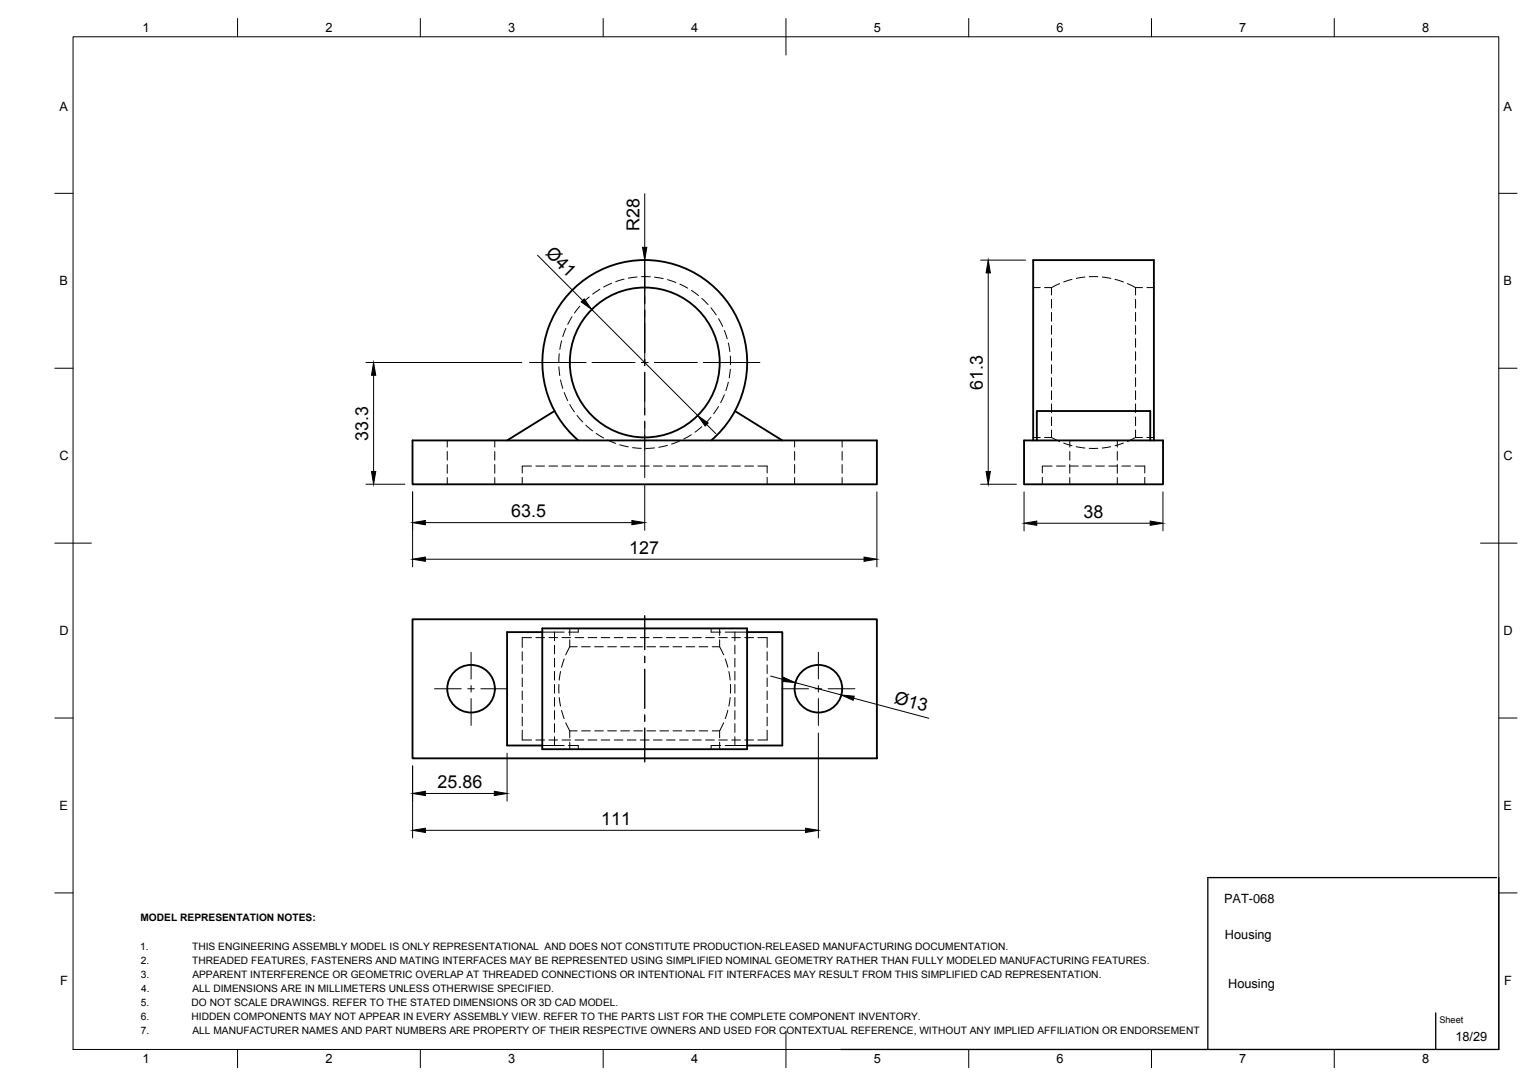
ISO-10303-21;
HEADER;
/* Generated by software containing ST-Developer
 * from STEP Tools, Inc. (www.steptools.com) 
 */

FILE_DESCRIPTION(
/* description */ ('Line shaft on three pillow blocks'),
/* implementation_level */ '2;1');

FILE_NAME(
/* name */ 'Housing.step',
/* time_stamp */ '2026-10-27T10:49:19-07:00',
/* author */ (''),
/* organization */ (''),
/* preprocessor_version */ 'ST-DEVELOPER v20.2',
/* originating_system */ 'Autodesk Translation Framework v15.17.0.0',
/* authorisation */ '');

FILE_SCHEMA (('AUTOMOTIVE_DESIGN { 1 0 10303 214 3 1 1 }'));
ENDSEC;

DATA;
#10=MECHANICAL_DESIGN_GEOMETRIC_PRESENTATION_REPRESENTATION('',(#351),#8377);
#263=SPHERICAL_SURFACE('',#4833,2.35);
#297=SHAPE_REPRESENTATION_RELATIONSHIP('SRR','None',#8513,#324);
#324=ADVANCED_BREP_SHAPE_REPRESENTATION('',(#378),#8362);
#351=STYLED_ITEM('',(#8697),#378);
#378=MANIFOLD_SOLID_BREP('Body1',#4338);
#430=FACE_BOUND('',#1041,.T.);
#431=FACE_BOUND('',#1042,.T.);
#432=FACE_BOUND('',#1050,.T.);
#433=FACE_BOUND('',#1051,.T.);
#434=FACE_BOUND('',#1052,.T.);
#435=FACE_BOUND('',#1055,.T.);
#436=FACE_BOUND('',#1057,.T.);
#437=FACE_BOUND('',#1070,.T.);
#438=FACE_BOUND('',#1071,.T.);
#439=FACE_BOUND('',#1072,.T.);
#547=PLANE('',#4835);
#548=PLANE('',#4837);
#549=PLANE('',#4839);
#550=PLANE('',#4841);
#551=PLANE('',#4842);
#552=PLANE('',#4844);
#553=PLANE('',#4845);
#554=PLANE('',#4851);
#555=PLANE('',#4852);
#556=PLANE('',#4853);
#557=PLANE('',#4854);
#558=PLANE('',#4855);
#559=PLANE('',#4856);
#560=PLANE('',#4857);
#561=PLANE('',#4862);
#562=PLANE('',#4863);
#563=PLANE('',#4864);
#564=PLANE('',#4865);
#565=PLANE('',#4866);
#747=FACE_OUTER_BOUND('',#1038,.T.);
#748=FACE_OUTER_BOUND('',#1039,.T.);
#749=FACE_OUTER_BOUND('',#1040,.T.);
#750=FACE_OUTER_BOUND('',#1043,.T.);
#751=FACE_OUTER_BOUND('',#1044,.T.);
#752=FACE_OUTER_BOUND('',#1045,.T.);
#753=FACE_OUTER_BOUND('',#1046,.T.);
#754=FACE_OUTER_BOUND('',#1047,.T.);
#755=FACE_OUTER_BOUND('',#1048,.T.);
#756=FACE_OUTER_BOUND('',#1049,.T.);
#757=FACE_OUTER_BOUND('',#1053,.T.);
#758=FACE_OUTER_BOUND('',#1054,.T.);
#759=FACE_OUTER_BOUND('',#1056,.T.);
#760=FACE_OUTER_BOUND('',#1058,.T.);
#761=FACE_OUTER_BOUND('',#1059,.T.);
#762=FACE_OUTER_BOUND('',#1060,.T.);
#763=FACE_OUTER_BOUND('',#1061,.T.);
#764=FACE_OUTER_BOUND('',#1062,.T.);
#765=FACE_OUTER_BOUND('',#1063,.T.);
#766=FACE_OUTER_BOUND('',#1064,.T.);
#767=FACE_OUTER_BOUND('',#1065,.T.);
#768=FACE_OUTER_BOUND('',#1066,.T.);
#769=FACE_OUTER_BOUND('',#1067,.T.);
#770=FACE_OUTER_BOUND('',#1068,.T.);
#771=FACE_OUTER_BOUND('',#1069,.T.);
#1038=EDGE_LOOP('',(#3301,#3302,#3303,#3304));
#1039=EDGE_LOOP('',(#3305,#3306,#3307,#3308));
#1040=EDGE_LOOP('',(#3309,#3310));
#1041=EDGE_LOOP('',(#3311));
#1042=EDGE_LOOP('',(#3312));
#1043=EDGE_LOOP('',(#3313,#3314,#3315));
#1044=EDGE_LOOP('',(#3316,#3317,#3318));
#1045=EDGE_LOOP('',(#3319,#3320,#3321));
#1046=EDGE_LOOP('',(#3322,#3323,#3324,#3325));
#1047=EDGE_LOOP('',(#3326,#3327,#3328));
#1048=EDGE_LOOP('',(#3329,#3330,#3331,#3332));
#1049=EDGE_LOOP('',(#3333,#3334,#3335,#3336));
#1050=EDGE_LOOP('',(#3337));
#1051=EDGE_LOOP('',(#3338));
#1052=EDGE_LOOP('',(#3339,#3340,#3341,#3342,#3343,#3344,#3345,#3346,#3347,
#3348,#3349,#3350));
#1053=EDGE_LOOP('',(#3351,#3352,#3353,#3354,#3355,#3356,#3357,#3358,#3359,
#3360,#3361,#3362));
#1054=EDGE_LOOP('',(#3363,#3364));
#1055=EDGE_LOOP('',(#3365));
#1056=EDGE_LOOP('',(#3366,#3367));
#1057=EDGE_LOOP('',(#3368));
#1058=EDGE_LOOP('',(#3369,#3370,#3371,#3372));
#1059=EDGE_LOOP('',(#3373,#3374,#3375,#3376));
#1060=EDGE_LOOP('',(#3377,#3378,#3379,#3380));
#1061=EDGE_LOOP('',(#3381,#3382,#3383,#3384));
#1062=EDGE_LOOP('',(#3385,#3386,#3387,#3388));
#1063=EDGE_LOOP('',(#3389,#3390,#3391,#3392));
#1064=EDGE_LOOP('',(#3393,#3394,#3395,#3396));
#1065=EDGE_LOOP('',(#3397,#3398,#3399,#3400));
#1066=EDGE_LOOP('',(#3401,#3402,#3403,#3404));
#1067=EDGE_LOOP('',(#3405,#3406,#3407,#3408));
#1068=EDGE_LOOP('',(#3409,#3410,#3411,#3412));
#1069=EDGE_LOOP('',(#3413,#3414,#3415,#3416));
#1070=EDGE_LOOP('',(#3417,#3418,#3419,#3420));
#1071=EDGE_LOOP('',(#3421));
#1072=EDGE_LOOP('',(#3422));
#1367=LINE('',#6871,#1694);
#1368=LINE('',#6877,#1695);
#1369=LINE('',#6886,#1696);
#1370=LINE('',#6888,#1697);
#1371=LINE('',#6893,#1698);
#1372=LINE('',#6896,#1699);
#1373=LINE('',#6900,#1700);
#1374=LINE('',#6903,#1701);
#1375=LINE('',#6905,#1702);
#1376=LINE('',#6906,#1703);
#1377=LINE('',#6910,#1704);
#1378=LINE('',#6912,#1705);
#1379=LINE('',#6915,#1706);
#1380=LINE('',#6916,#1707);
#1381=LINE('',#6920,#1708);
#1382=LINE('',#6922,#1709);
#1383=LINE('',#6924,#1710);
#1384=LINE('',#6925,#1711);
#1385=LINE('',#6931,#1712);
#1386=LINE('',#6933,#1713);
#1387=LINE('',#6934,#1714);
#1388=LINE('',#6936,#1715);
#1389=LINE('',#6938,#1716);
#1390=LINE('',#6939,#1717);
#1391=LINE('',#6948,#1718);
#1392=LINE('',#6950,#1719);
#1393=LINE('',#6952,#1720);
#1394=LINE('',#6953,#1721);
#1395=LINE('',#6956,#1722);
#1396=LINE('',#6958,#1723);
#1397=LINE('',#6959,#1724);
#1398=LINE('',#6962,#1725);
#1399=LINE('',#6964,#1726);
#1400=LINE('',#6965,#1727);
#1401=LINE('',#6967,#1728);
#1402=LINE('',#6968,#1729);
#1403=LINE('',#6973,#1730);
#1404=LINE('',#6977,#1731);
#1405=LINE('',#6981,#1732);
#1406=LINE('',#6982,#1733);
#1407=LINE('',#6983,#1734);
#1408=LINE('',#6986,#1735);
#1409=LINE('',#6987,#1736);
#1410=LINE('',#6990,#1737);
#1411=LINE('',#6991,#1738);
#1412=LINE('',#6993,#1739);
#1694=VECTOR('',#5612,2.05);
#1695=VECTOR('',#5619,2.05);
#1696=VECTOR('',#5628,1.);
#1697=VECTOR('',#5629,1.);
#1698=VECTOR('',#5634,1.);
#1699=VECTOR('',#5637,1.);
#1700=VECTOR('',#5640,1.);
#1701=VECTOR('',#5643,1.);
#1702=VECTOR('',#5646,1.);
#1703=VECTOR('',#5647,1.);
#1704=VECTOR('',#5650,1.);
#1705=VECTOR('',#5651,1.);
#1706=VECTOR('',#5656,1.);
#1707=VECTOR('',#5657,1.);
#1708=VECTOR('',#5660,1.);
#1709=VECTOR('',#5661,1.);
#1710=VECTOR('',#5662,1.);
#1711=VECTOR('',#5663,1.);
#1712=VECTOR('',#5668,1.);
#1713=VECTOR('',#5669,1.);
#1714=VECTOR('',#5670,1.);
#1715=VECTOR('',#5671,1.);
#1716=VECTOR('',#5672,1.);
#1717=VECTOR('',#5673,1.);
#1718=VECTOR('',#5686,1.);
#1719=VECTOR('',#5687,1.);
#1720=VECTOR('',#5688,1.);
#1721=VECTOR('',#5689,1.);
#1722=VECTOR('',#5692,1.);
#1723=VECTOR('',#5693,1.);
#1724=VECTOR('',#5694,1.);
#1725=VECTOR('',#5697,1.);
#1726=VECTOR('',#5698,1.);
#1727=VECTOR('',#5699,1.);
#1728=VECTOR('',#5702,1.);
#1729=VECTOR('',#5703,1.);
#1730=VECTOR('',#5710,0.65);
#1731=VECTOR('',#5715,0.65);
#1732=VECTOR('',#5718,1.);
#1733=VECTOR('',#5719,1.);
#1734=VECTOR('',#5720,1.);
#1735=VECTOR('',#5723,1.);
#1736=VECTOR('',#5724,1.);
#1737=VECTOR('',#5727,1.);
#1738=VECTOR('',#5728,1.);
#1739=VECTOR('',#5731,1.);
#1973=CIRCLE('',#4828,2.05);
#1974=CIRCLE('',#4829,2.05);
#1975=CIRCLE('',#4831,2.05);
#1976=CIRCLE('',#4832,2.05);
#1977=CIRCLE('',#4834,2.35);
#1978=CIRCLE('',#4836,2.8);
#1979=CIRCLE('',#4838,2.8);
#1980=CIRCLE('',#4840,2.8);
#1981=CIRCLE('',#4843,2.8);
#1982=CIRCLE('',#4846,0.65);
#1983=CIRCLE('',#4847,0.65);
#1984=CIRCLE('',#4849,2.8);
#1985=CIRCLE('',#4850,2.8);
#1986=CIRCLE('',#4859,0.65);
#1987=CIRCLE('',#4861,0.65);
#2184=VERTEX_POINT('',#6868);
#2185=VERTEX_POINT('',#6870);
#2186=VERTEX_POINT('',#6874);
#2187=VERTEX_POINT('',#6876);
#2188=VERTEX_POINT('',#6880);
#2189=VERTEX_POINT('',#6881);
#2190=VERTEX_POINT('',#6884);
#2191=VERTEX_POINT('',#6885);
#2192=VERTEX_POINT('',#6887);
#2193=VERTEX_POINT('',#6891);
#2194=VERTEX_POINT('',#6892);
#2195=VERTEX_POINT('',#6894);
#2196=VERTEX_POINT('',#6898);
#2197=VERTEX_POINT('',#6899);
#2198=VERTEX_POINT('',#6901);
#2199=VERTEX_POINT('',#6908);
#2200=VERTEX_POINT('',#6909);
#2201=VERTEX_POINT('',#6911);
#2202=VERTEX_POINT('',#6918);
#2203=VERTEX_POINT('',#6919);
#2204=VERTEX_POINT('',#6921);
#2205=VERTEX_POINT('',#6923);
#2206=VERTEX_POINT('',#6926);
#2207=VERTEX_POINT('',#6928);
#2208=VERTEX_POINT('',#6930);
#2209=VERTEX_POINT('',#6932);
#2210=VERTEX_POINT('',#6935);
#2211=VERTEX_POINT('',#6937);
#2212=VERTEX_POINT('',#6946);
#2213=VERTEX_POINT('',#6947);
#2214=VERTEX_POINT('',#6949);
#2215=VERTEX_POINT('',#6951);
#2216=VERTEX_POINT('',#6955);
#2217=VERTEX_POINT('',#6957);
#2218=VERTEX_POINT('',#6961);
#2219=VERTEX_POINT('',#6963);
#2220=VERTEX_POINT('',#6971);
#2221=VERTEX_POINT('',#6975);
#2222=VERTEX_POINT('',#6979);
#2223=VERTEX_POINT('',#6980);
#2224=VERTEX_POINT('',#6985);
#2225=VERTEX_POINT('',#6989);
#2599=EDGE_CURVE('',#2184,#2184,#1973,.T.);
#2600=EDGE_CURVE('',#2184,#2185,#1367,.T.);
#2601=EDGE_CURVE('',#2185,#2185,#1974,.T.);
#2602=EDGE_CURVE('',#2186,#2186,#1975,.T.);
#2603=EDGE_CURVE('',#2186,#2187,#1368,.T.);
#2604=EDGE_CURVE('',#2187,#2187,#1976,.T.);
#2605=EDGE_CURVE('',#2188,#2189,#1977,.T.);
#2606=EDGE_CURVE('',#2190,#2191,#1369,.T.);
#2607=EDGE_CURVE('',#2190,#2192,#1370,.T.);
#2608=EDGE_CURVE('',#2191,#2192,#1978,.T.);
#2609=EDGE_CURVE('',#2193,#2194,#1371,.T.);
#2610=EDGE_CURVE('',#2195,#2193,#1979,.T.);
#2611=EDGE_CURVE('',#2195,#2194,#1372,.T.);
#2612=EDGE_CURVE('',#2196,#2197,#1373,.T.);
#2613=EDGE_CURVE('',#2198,#2196,#1980,.T.);
#2614=EDGE_CURVE('',#2198,#2197,#1374,.T.);
#2615=EDGE_CURVE('',#2197,#2190,#1375,.T.);
#2616=EDGE_CURVE('',#2192,#2198,#1376,.T.);
#2617=EDGE_CURVE('',#2199,#2200,#1377,.T.);
#2618=EDGE_CURVE('',#2199,#2201,#1378,.T.);
#2619=EDGE_CURVE('',#2200,#2201,#1981,.T.);
#2620=EDGE_CURVE('',#2194,#2199,#1379,.T.);
#2621=EDGE_CURVE('',#2201,#2195,#1380,.T.);
#2622=EDGE_CURVE('',#2202,#2203,#1381,.T.);
#2623=EDGE_CURVE('',#2203,#2204,#1382,.T.);
#2624=EDGE_CURVE('',#2204,#2205,#1383,.T.);
#2625=EDGE_CURVE('',#2205,#2202,#1384,.T.);
#2626=EDGE_CURVE('',#2206,#2206,#1982,.T.);
#2627=EDGE_CURVE('',#2207,#2207,#1983,.T.);
#2628=EDGE_CURVE('',#2200,#2208,#1385,.T.);
#2629=EDGE_CURVE('',#2208,#2209,#1386,.T.);
#2630=EDGE_CURVE('',#2209,#2196,#1387,.T.);
#2631=EDGE_CURVE('',#2191,#2210,#1388,.T.);
#2632=EDGE_CURVE('',#2210,#2211,#1389,.T.);
#2633=EDGE_CURVE('',#2211,#2193,#1390,.T.);
#2634=EDGE_CURVE('',#2210,#2211,#1984,.T.);
#2635=EDGE_CURVE('',#2208,#2209,#1985,.T.);
#2636=EDGE_CURVE('',#2212,#2213,#1391,.T.);
#2637=EDGE_CURVE('',#2212,#2214,#1392,.T.);
#2638=EDGE_CURVE('',#2214,#2215,#1393,.T.);
#2639=EDGE_CURVE('',#2213,#2215,#1394,.T.);
#2640=EDGE_CURVE('',#2216,#2212,#1395,.T.);
#2641=EDGE_CURVE('',#2216,#2217,#1396,.T.);
#2642=EDGE_CURVE('',#2217,#2214,#1397,.T.);
#2643=EDGE_CURVE('',#2218,#2216,#1398,.T.);
#2644=EDGE_CURVE('',#2218,#2219,#1399,.T.);
#2645=EDGE_CURVE('',#2219,#2217,#1400,.T.);
#2646=EDGE_CURVE('',#2213,#2218,#1401,.T.);
#2647=EDGE_CURVE('',#2215,#2219,#1402,.T.);
#2648=EDGE_CURVE('',#2220,#2220,#1986,.T.);
#2649=EDGE_CURVE('',#2220,#2207,#1403,.T.);
#2650=EDGE_CURVE('',#2221,#2221,#1987,.T.);
#2651=EDGE_CURVE('',#2221,#2206,#1404,.T.);
#2652=EDGE_CURVE('',#2222,#2223,#1405,.T.);
#2653=EDGE_CURVE('',#2223,#2202,#1406,.T.);
#2654=EDGE_CURVE('',#2222,#2205,#1407,.T.);
#2655=EDGE_CURVE('',#2224,#2222,#1408,.T.);
#2656=EDGE_CURVE('',#2224,#2204,#1409,.T.);
#2657=EDGE_CURVE('',#2225,#2224,#1410,.T.);
#2658=EDGE_CURVE('',#2225,#2203,#1411,.T.);
#2659=EDGE_CURVE('',#2223,#2225,#1412,.T.);
#3301=ORIENTED_EDGE('',*,*,#2599,.F.);
#3302=ORIENTED_EDGE('',*,*,#2600,.T.);
#3303=ORIENTED_EDGE('',*,*,#2601,.F.);
#3304=ORIENTED_EDGE('',*,*,#2600,.F.);
#3305=ORIENTED_EDGE('',*,*,#2602,.F.);
#3306=ORIENTED_EDGE('',*,*,#2603,.T.);
#3307=ORIENTED_EDGE('',*,*,#2604,.F.);
#3308=ORIENTED_EDGE('',*,*,#2603,.F.);
#3309=ORIENTED_EDGE('',*,*,#2605,.T.);
#3310=ORIENTED_EDGE('',*,*,#2605,.F.);
#3311=ORIENTED_EDGE('',*,*,#2602,.T.);
#3312=ORIENTED_EDGE('',*,*,#2601,.T.);
#3313=ORIENTED_EDGE('',*,*,#2606,.F.);
#3314=ORIENTED_EDGE('',*,*,#2607,.T.);
#3315=ORIENTED_EDGE('',*,*,#2608,.F.);
#3316=ORIENTED_EDGE('',*,*,#2609,.F.);
#3317=ORIENTED_EDGE('',*,*,#2610,.F.);
#3318=ORIENTED_EDGE('',*,*,#2611,.T.);
#3319=ORIENTED_EDGE('',*,*,#2612,.F.);
#3320=ORIENTED_EDGE('',*,*,#2613,.F.);
#3321=ORIENTED_EDGE('',*,*,#2614,.T.);
#3322=ORIENTED_EDGE('',*,*,#2615,.F.);
#3323=ORIENTED_EDGE('',*,*,#2614,.F.);
#3324=ORIENTED_EDGE('',*,*,#2616,.F.);
#3325=ORIENTED_EDGE('',*,*,#2607,.F.);
#3326=ORIENTED_EDGE('',*,*,#2617,.F.);
#3327=ORIENTED_EDGE('',*,*,#2618,.T.);
#3328=ORIENTED_EDGE('',*,*,#2619,.F.);
#3329=ORIENTED_EDGE('',*,*,#2620,.F.);
#3330=ORIENTED_EDGE('',*,*,#2611,.F.);
#3331=ORIENTED_EDGE('',*,*,#2621,.F.);
#3332=ORIENTED_EDGE('',*,*,#2618,.F.);
#3333=ORIENTED_EDGE('',*,*,#2622,.T.);
#3334=ORIENTED_EDGE('',*,*,#2623,.T.);
#3335=ORIENTED_EDGE('',*,*,#2624,.T.);
#3336=ORIENTED_EDGE('',*,*,#2625,.T.);
#3337=ORIENTED_EDGE('',*,*,#2626,.T.);
#3338=ORIENTED_EDGE('',*,*,#2627,.T.);
#3339=ORIENTED_EDGE('',*,*,#2609,.T.);
#3340=ORIENTED_EDGE('',*,*,#2620,.T.);
#3341=ORIENTED_EDGE('',*,*,#2617,.T.);
#3342=ORIENTED_EDGE('',*,*,#2628,.T.);
#3343=ORIENTED_EDGE('',*,*,#2629,.T.);
#3344=ORIENTED_EDGE('',*,*,#2630,.T.);
#3345=ORIENTED_EDGE('',*,*,#2612,.T.);
#3346=ORIENTED_EDGE('',*,*,#2615,.T.);
#3347=ORIENTED_EDGE('',*,*,#2606,.T.);
#3348=ORIENTED_EDGE('',*,*,#2631,.T.);
#3349=ORIENTED_EDGE('',*,*,#2632,.T.);
#3350=ORIENTED_EDGE('',*,*,#2633,.T.);
#3351=ORIENTED_EDGE('',*,*,#2610,.T.);
#3352=ORIENTED_EDGE('',*,*,#2633,.F.);
#3353=ORIENTED_EDGE('',*,*,#2634,.F.);
#3354=ORIENTED_EDGE('',*,*,#2631,.F.);
#3355=ORIENTED_EDGE('',*,*,#2608,.T.);
#3356=ORIENTED_EDGE('',*,*,#2616,.T.);
#3357=ORIENTED_EDGE('',*,*,#2613,.T.);
#3358=ORIENTED_EDGE('',*,*,#2630,.F.);
#3359=ORIENTED_EDGE('',*,*,#2635,.F.);
#3360=ORIENTED_EDGE('',*,*,#2628,.F.);
#3361=ORIENTED_EDGE('',*,*,#2619,.T.);
#3362=ORIENTED_EDGE('',*,*,#2621,.T.);
#3363=ORIENTED_EDGE('',*,*,#2629,.F.);
#3364=ORIENTED_EDGE('',*,*,#2635,.T.);
#3365=ORIENTED_EDGE('',*,*,#2599,.T.);
#3366=ORIENTED_EDGE('',*,*,#2632,.F.);
#3367=ORIENTED_EDGE('',*,*,#2634,.T.);
#3368=ORIENTED_EDGE('',*,*,#2604,.T.);
#3369=ORIENTED_EDGE('',*,*,#2636,.F.);
#3370=ORIENTED_EDGE('',*,*,#2637,.T.);
#3371=ORIENTED_EDGE('',*,*,#2638,.T.);
#3372=ORIENTED_EDGE('',*,*,#2639,.F.);
#3373=ORIENTED_EDGE('',*,*,#2640,.F.);
#3374=ORIENTED_EDGE('',*,*,#2641,.T.);
#3375=ORIENTED_EDGE('',*,*,#2642,.T.);
#3376=ORIENTED_EDGE('',*,*,#2637,.F.);
#3377=ORIENTED_EDGE('',*,*,#2643,.F.);
#3378=ORIENTED_EDGE('',*,*,#2644,.T.);
#3379=ORIENTED_EDGE('',*,*,#2645,.T.);
#3380=ORIENTED_EDGE('',*,*,#2641,.F.);
#3381=ORIENTED_EDGE('',*,*,#2646,.F.);
#3382=ORIENTED_EDGE('',*,*,#2639,.T.);
#3383=ORIENTED_EDGE('',*,*,#2647,.T.);
#3384=ORIENTED_EDGE('',*,*,#2644,.F.);
#3385=ORIENTED_EDGE('',*,*,#2647,.F.);
#3386=ORIENTED_EDGE('',*,*,#2638,.F.);
#3387=ORIENTED_EDGE('',*,*,#2642,.F.);
#3388=ORIENTED_EDGE('',*,*,#2645,.F.);
#3389=ORIENTED_EDGE('',*,*,#2648,.F.);
#3390=ORIENTED_EDGE('',*,*,#2649,.T.);
#3391=ORIENTED_EDGE('',*,*,#2627,.F.);
#3392=ORIENTED_EDGE('',*,*,#2649,.F.);
#3393=ORIENTED_EDGE('',*,*,#2650,.F.);
#3394=ORIENTED_EDGE('',*,*,#2651,.T.);
#3395=ORIENTED_EDGE('',*,*,#2626,.F.);
#3396=ORIENTED_EDGE('',*,*,#2651,.F.);
#3397=ORIENTED_EDGE('',*,*,#2652,.T.);
#3398=ORIENTED_EDGE('',*,*,#2653,.T.);
#3399=ORIENTED_EDGE('',*,*,#2625,.F.);
#3400=ORIENTED_EDGE('',*,*,#2654,.F.);
#3401=ORIENTED_EDGE('',*,*,#2655,.T.);
#3402=ORIENTED_EDGE('',*,*,#2654,.T.);
#3403=ORIENTED_EDGE('',*,*,#2624,.F.);
#3404=ORIENTED_EDGE('',*,*,#2656,.F.);
#3405=ORIENTED_EDGE('',*,*,#2657,.T.);
#3406=ORIENTED_EDGE('',*,*,#2656,.T.);
#3407=ORIENTED_EDGE('',*,*,#2623,.F.);
#3408=ORIENTED_EDGE('',*,*,#2658,.F.);
#3409=ORIENTED_EDGE('',*,*,#2659,.T.);
#3410=ORIENTED_EDGE('',*,*,#2658,.T.);
#3411=ORIENTED_EDGE('',*,*,#2622,.F.);
#3412=ORIENTED_EDGE('',*,*,#2653,.F.);
#3413=ORIENTED_EDGE('',*,*,#2659,.F.);
#3414=ORIENTED_EDGE('',*,*,#2652,.F.);
#3415=ORIENTED_EDGE('',*,*,#2655,.F.);
#3416=ORIENTED_EDGE('',*,*,#2657,.F.);
#3417=ORIENTED_EDGE('',*,*,#2636,.T.);
#3418=ORIENTED_EDGE('',*,*,#2646,.T.);
#3419=ORIENTED_EDGE('',*,*,#2643,.T.);
#3420=ORIENTED_EDGE('',*,*,#2640,.T.);
#3421=ORIENTED_EDGE('',*,*,#2648,.T.);
#3422=ORIENTED_EDGE('',*,*,#2650,.T.);
#4031=CYLINDRICAL_SURFACE('',#4827,2.05);
#4032=CYLINDRICAL_SURFACE('',#4830,2.05);
#4033=CYLINDRICAL_SURFACE('',#4848,2.8);
#4034=CYLINDRICAL_SURFACE('',#4858,0.65);
#4035=CYLINDRICAL_SURFACE('',#4860,0.65);
#4165=ADVANCED_FACE('',(#747),#4031,.F.);
#4166=ADVANCED_FACE('',(#748),#4032,.F.);
#4167=ADVANCED_FACE('',(#749,#430,#431),#263,.F.);
#4168=ADVANCED_FACE('',(#750),#547,.T.);
#4169=ADVANCED_FACE('',(#751),#548,.T.);
#4170=ADVANCED_FACE('',(#752),#549,.T.);
#4171=ADVANCED_FACE('',(#753),#550,.T.);
#4172=ADVANCED_FACE('',(#754),#551,.T.);
#4173=ADVANCED_FACE('',(#755),#552,.T.);
#4174=ADVANCED_FACE('',(#756,#432,#433,#434),#553,.T.);
#4175=ADVANCED_FACE('',(#757),#4033,.T.);
#4176=ADVANCED_FACE('',(#758,#435),#554,.F.);
#4177=ADVANCED_FACE('',(#759,#436),#555,.T.);
#4178=ADVANCED_FACE('',(#760),#556,.F.);
#4179=ADVANCED_FACE('',(#761),#557,.F.);
#4180=ADVANCED_FACE('',(#762),#558,.F.);
#4181=ADVANCED_FACE('',(#763),#559,.F.);
#4182=ADVANCED_FACE('',(#764),#560,.F.);
#4183=ADVANCED_FACE('',(#765),#4034,.F.);
#4184=ADVANCED_FACE('',(#766),#4035,.F.);
#4185=ADVANCED_FACE('',(#767),#561,.T.);
#4186=ADVANCED_FACE('',(#768),#562,.T.);
#4187=ADVANCED_FACE('',(#769),#563,.T.);
#4188=ADVANCED_FACE('',(#770),#564,.T.);
#4189=ADVANCED_FACE('',(#771,#437,#438,#439),#565,.F.);
#4338=CLOSED_SHELL('',(#4165,#4166,#4167,#4168,#4169,#4170,#4171,#4172,
#4173,#4174,#4175,#4176,#4177,#4178,#4179,#4180,#4181,#4182,#4183,#4184,
#4185,#4186,#4187,#4188,#4189));
#4826=AXIS2_PLACEMENT_3D('',#6866,#5606,#5607);
#4827=AXIS2_PLACEMENT_3D('',#6867,#5608,#5609);
#4828=AXIS2_PLACEMENT_3D('',#6869,#5610,#5611);
#4829=AXIS2_PLACEMENT_3D('',#6872,#5613,#5614);
#4830=AXIS2_PLACEMENT_3D('',#6873,#5615,#5616);
#4831=AXIS2_PLACEMENT_3D('',#6875,#5617,#5618);
#4832=AXIS2_PLACEMENT_3D('',#6878,#5620,#5621);
#4833=AXIS2_PLACEMENT_3D('',#6879,#5622,#5623);
#4834=AXIS2_PLACEMENT_3D('',#6882,#5624,#5625);
#4835=AXIS2_PLACEMENT_3D('',#6883,#5626,#5627);
#4836=AXIS2_PLACEMENT_3D('',#6889,#5630,#5631);
#4837=AXIS2_PLACEMENT_3D('',#6890,#5632,#5633);
#4838=AXIS2_PLACEMENT_3D('',#6895,#5635,#5636);
#4839=AXIS2_PLACEMENT_3D('',#6897,#5638,#5639);
#4840=AXIS2_PLACEMENT_3D('',#6902,#5641,#5642);
#4841=AXIS2_PLACEMENT_3D('',#6904,#5644,#5645);
#4842=AXIS2_PLACEMENT_3D('',#6907,#5648,#5649);
#4843=AXIS2_PLACEMENT_3D('',#6913,#5652,#5653);
#4844=AXIS2_PLACEMENT_3D('',#6914,#5654,#5655);
#4845=AXIS2_PLACEMENT_3D('',#6917,#5658,#5659);
#4846=AXIS2_PLACEMENT_3D('',#6927,#5664,#5665);
#4847=AXIS2_PLACEMENT_3D('',#6929,#5666,#5667);
#4848=AXIS2_PLACEMENT_3D('',#6940,#5674,#5675);
#4849=AXIS2_PLACEMENT_3D('',#6941,#5676,#5677);
#4850=AXIS2_PLACEMENT_3D('',#6942,#5678,#5679);
#4851=AXIS2_PLACEMENT_3D('',#6943,#5680,#5681);
#4852=AXIS2_PLACEMENT_3D('',#6944,#5682,#5683);
#4853=AXIS2_PLACEMENT_3D('',#6945,#5684,#5685);
#4854=AXIS2_PLACEMENT_3D('',#6954,#5690,#5691);
#4855=AXIS2_PLACEMENT_3D('',#6960,#5695,#5696);
#4856=AXIS2_PLACEMENT_3D('',#6966,#5700,#5701);
#4857=AXIS2_PLACEMENT_3D('',#6969,#5704,#5705);
#4858=AXIS2_PLACEMENT_3D('',#6970,#5706,#5707);
#4859=AXIS2_PLACEMENT_3D('',#6972,#5708,#5709);
#4860=AXIS2_PLACEMENT_3D('',#6974,#5711,#5712);
#4861=AXIS2_PLACEMENT_3D('',#6976,#5713,#5714);
#4862=AXIS2_PLACEMENT_3D('',#6978,#5716,#5717);
#4863=AXIS2_PLACEMENT_3D('',#6984,#5721,#5722);
#4864=AXIS2_PLACEMENT_3D('',#6988,#5725,#5726);
#4865=AXIS2_PLACEMENT_3D('',#6992,#5729,#5730);
#4866=AXIS2_PLACEMENT_3D('',#6994,#5732,#5733);
#5606=DIRECTION('axis',(0.,0.,1.));
#5607=DIRECTION('refdir',(1.,0.,0.));
#5608=DIRECTION('center_axis',(0.,1.,0.));
#5609=DIRECTION('ref_axis',(1.,0.,0.));
#5610=DIRECTION('center_axis',(0.,1.,0.));
#5611=DIRECTION('ref_axis',(1.,0.,0.));
#5612=DIRECTION('',(0.,1.,0.));
#5613=DIRECTION('center_axis',(0.,-1.,0.));
#5614=DIRECTION('ref_axis',(1.,0.,0.));
#5615=DIRECTION('center_axis',(0.,1.,0.));
#5616=DIRECTION('ref_axis',(1.,0.,0.));
#5617=DIRECTION('center_axis',(0.,1.,0.));
#5618=DIRECTION('ref_axis',(1.,0.,0.));
#5619=DIRECTION('',(0.,1.,0.));
#5620=DIRECTION('center_axis',(0.,-1.,0.));
#5621=DIRECTION('ref_axis',(1.,0.,0.));
#5622=DIRECTION('center_axis',(6.12323399573677E-17,0.,1.));
#5623=DIRECTION('ref_axis',(1.,0.,0.));
#5624=DIRECTION('center_axis',(-1.22464679914735E-16,1.,0.));
#5625=DIRECTION('ref_axis',(-1.,-1.22464679914735E-16,0.));
#5626=DIRECTION('center_axis',(0.,1.,0.));
#5627=DIRECTION('ref_axis',(0.,0.,1.));
#5628=DIRECTION('',(1.,0.,0.));
#5629=DIRECTION('',(0.850265146687862,0.,0.526354614616295));
#5630=DIRECTION('center_axis',(0.,1.,0.));
#5631=DIRECTION('ref_axis',(1.,0.,0.));
#5632=DIRECTION('center_axis',(0.,1.,0.));
#5633=DIRECTION('ref_axis',(0.,0.,1.));
#5634=DIRECTION('',(1.,0.,0.));
#5635=DIRECTION('center_axis',(0.,1.,0.));
#5636=DIRECTION('ref_axis',(1.,0.,0.));
#5637=DIRECTION('',(0.850265146687862,0.,-0.526354614616295));
#5638=DIRECTION('center_axis',(0.,-1.,0.));
#5639=DIRECTION('ref_axis',(0.,0.,-1.));
#5640=DIRECTION('',(-1.,0.,0.));
#5641=DIRECTION('center_axis',(0.,-1.,0.));
#5642=DIRECTION('ref_axis',(1.,0.,0.));
#5643=DIRECTION('',(-0.850265146687862,0.,-0.526354614616295));
#5644=DIRECTION('center_axis',(-0.526354614616295,0.,0.850265146687862));
#5645=DIRECTION('ref_axis',(0.850265146687862,0.,0.526354614616295));
#5646=DIRECTION('',(0.,1.,0.));
#5647=DIRECTION('',(0.,-1.,0.));
#5648=DIRECTION('center_axis',(0.,-1.,0.));
#5649=DIRECTION('ref_axis',(0.,0.,-1.));
#5650=DIRECTION('',(-1.,0.,0.));
#5651=DIRECTION('',(-0.850265146687862,0.,0.526354614616295));
#5652=DIRECTION('center_axis',(0.,-1.,0.));
#5653=DIRECTION('ref_axis',(1.,0.,0.));
#5654=DIRECTION('center_axis',(0.526354614616295,0.,0.850265146687862));
#5655=DIRECTION('ref_axis',(0.850265146687862,0.,-0.526354614616295));
#5656=DIRECTION('',(0.,-1.,0.));
#5657=DIRECTION('',(0.,1.,0.));
#5658=DIRECTION('center_axis',(0.,0.,1.));
#5659=DIRECTION('ref_axis',(1.,0.,0.));
#5660=DIRECTION('',(0.,-1.,0.));
#5661=DIRECTION('',(1.,0.,0.));
#5662=DIRECTION('',(0.,1.,0.));
#5663=DIRECTION('',(-1.,0.,0.));
#5664=DIRECTION('center_axis',(0.,0.,-1.));
#5665=DIRECTION('ref_axis',(1.,0.,0.));
#5666=DIRECTION('center_axis',(0.,0.,-1.));
#5667=DIRECTION('ref_axis',(1.,0.,0.));
#5668=DIRECTION('',(0.,-1.,0.));
#5669=DIRECTION('',(-1.,0.,0.));
#5670=DIRECTION('',(0.,1.,0.));
#5671=DIRECTION('',(0.,1.,0.));
#5672=DIRECTION('',(1.,0.,0.));
#5673=DIRECTION('',(0.,-1.,0.));
#5674=DIRECTION('center_axis',(0.,1.,0.));
#5675=DIRECTION('ref_axis',(6.12323399573677E-17,0.,1.));
#5676=DIRECTION('center_axis',(0.,1.,0.));
#5677=DIRECTION('ref_axis',(1.,0.,0.));
#5678=DIRECTION('center_axis',(0.,-1.,0.));
#5679=DIRECTION('ref_axis',(1.,0.,0.));
#5680=DIRECTION('center_axis',(0.,1.,0.));
#5681=DIRECTION('ref_axis',(1.,0.,0.));
#5682=DIRECTION('center_axis',(0.,1.,0.));
#5683=DIRECTION('ref_axis',(1.,0.,0.));
#5684=DIRECTION('center_axis',(0.,1.,0.));
#5685=DIRECTION('ref_axis',(-1.,0.,0.));
#5686=DIRECTION('',(-1.,0.,0.));
#5687=DIRECTION('',(0.,0.,1.));
#5688=DIRECTION('',(-1.,0.,0.));
#5689=DIRECTION('',(0.,0.,1.));
#5690=DIRECTION('center_axis',(1.,0.,0.));
#5691=DIRECTION('ref_axis',(0.,1.,0.));
#5692=DIRECTION('',(0.,1.,0.));
#5693=DIRECTION('',(0.,0.,1.));
#5694=DIRECTION('',(0.,1.,0.));
#5695=DIRECTION('center_axis',(0.,-1.,0.));
#5696=DIRECTION('ref_axis',(1.,0.,0.));
#5697=DIRECTION('',(1.,0.,0.));
#5698=DIRECTION('',(0.,0.,1.));
#5699=DIRECTION('',(1.,0.,0.));
#5700=DIRECTION('center_axis',(-1.,0.,0.));
#5701=DIRECTION('ref_axis',(0.,-1.,0.));
#5702=DIRECTION('',(0.,-1.,0.));
#5703=DIRECTION('',(0.,-1.,0.));
#5704=DIRECTION('center_axis',(0.,0.,1.));
#5705=DIRECTION('ref_axis',(1.,0.,0.));
#5706=DIRECTION('center_axis',(0.,0.,1.));
#5707=DIRECTION('ref_axis',(1.,0.,0.));
#5708=DIRECTION('center_axis',(0.,0.,1.));
#5709=DIRECTION('ref_axis',(1.,0.,0.));
#5710=DIRECTION('',(0.,0.,1.));
#5711=DIRECTION('center_axis',(0.,0.,1.));
#5712=DIRECTION('ref_axis',(1.,0.,0.));
#5713=DIRECTION('center_axis',(0.,0.,1.));
#5714=DIRECTION('ref_axis',(1.,0.,0.));
#5715=DIRECTION('',(0.,0.,1.));
#5716=DIRECTION('center_axis',(0.,1.,0.));
#5717=DIRECTION('ref_axis',(-1.,0.,0.));
#5718=DIRECTION('',(-1.,0.,0.));
#5719=DIRECTION('',(0.,0.,1.));
#5720=DIRECTION('',(0.,0.,1.));
#5721=DIRECTION('center_axis',(1.,0.,0.));
#5722=DIRECTION('ref_axis',(0.,1.,0.));
#5723=DIRECTION('',(0.,1.,0.));
#5724=DIRECTION('',(0.,0.,1.));
#5725=DIRECTION('center_axis',(0.,-1.,0.));
#5726=DIRECTION('ref_axis',(1.,0.,0.));
#5727=DIRECTION('',(1.,0.,0.));
#5728=DIRECTION('',(0.,0.,1.));
#5729=DIRECTION('center_axis',(-1.,0.,0.));
#5730=DIRECTION('ref_axis',(0.,-1.,0.));
#5731=DIRECTION('',(0.,-1.,0.));
#5732=DIRECTION('center_axis',(0.,0.,1.));
#5733=DIRECTION('ref_axis',(1.,0.,0.));
#6866=CARTESIAN_POINT('',(0.,0.,0.));
#6867=CARTESIAN_POINT('Origin',(0.,0.,0.));
#6868=CARTESIAN_POINT('',(-2.05,-1.65,2.51052593825207E-16));
#6869=CARTESIAN_POINT('Origin',(0.,-1.65,0.));
#6870=CARTESIAN_POINT('',(-2.05,-1.14891252930761,-2.51052593825207E-16));
#6871=CARTESIAN_POINT('',(-2.05,0.,2.51052593825207E-16));
#6872=CARTESIAN_POINT('Origin',(0.,-1.14891252930761,0.));
#6873=CARTESIAN_POINT('Origin',(0.,0.,0.));
#6874=CARTESIAN_POINT('',(-2.05,1.14891252930761,2.51052593825207E-16));
#6875=CARTESIAN_POINT('Origin',(0.,1.14891252930761,0.));
#6876=CARTESIAN_POINT('',(-2.05,1.65,-2.51052593825207E-16));
#6877=CARTESIAN_POINT('',(-2.05,0.,2.51052593825207E-16));
#6878=CARTESIAN_POINT('Origin',(0.,1.65,0.));
#6879=CARTESIAN_POINT('Origin',(0.,0.,0.));
#6880=CARTESIAN_POINT('',(-1.43895998899814E-16,-1.76221774462768E-32,-2.35));
#6881=CARTESIAN_POINT('',(-1.43895998899814E-16,-1.76221774462768E-32,2.35));
#6882=CARTESIAN_POINT('Origin',(0.,0.,0.));
#6883=CARTESIAN_POINT('Origin',(0.,1.55,-1.49));
#6884=CARTESIAN_POINT('',(-3.76384615384615,1.55,-2.13));
#6885=CARTESIAN_POINT('',(-1.81744325908679,1.55,-2.13));
#6886=CARTESIAN_POINT('',(0.,1.55,-2.13));
#6887=CARTESIAN_POINT('',(-2.46585583768694,1.55,-1.32648218523477));
#6888=CARTESIAN_POINT('',(-1.68,1.55,-0.84));
#6889=CARTESIAN_POINT('Origin',(0.,1.55,0.));
#6890=CARTESIAN_POINT('Origin',(0.,1.55,-1.49));
#6891=CARTESIAN_POINT('',(1.81744325908679,1.55,-2.13));
#6892=CARTESIAN_POINT('',(3.76384615384615,1.55,-2.13));
#6893=CARTESIAN_POINT('',(0.,1.55,-2.13));
#6894=CARTESIAN_POINT('',(2.46585583768694,1.55,-1.32648218523477));
#6895=CARTESIAN_POINT('Origin',(0.,1.55,0.));
#6896=CARTESIAN_POINT('',(3.78,1.55,-2.14));
#6897=CARTESIAN_POINT('Origin',(0.,-1.55,-1.49));
#6898=CARTESIAN_POINT('',(-1.81744325908679,-1.55,-2.13));
#6899=CARTESIAN_POINT('',(-3.76384615384615,-1.55,-2.13));
#6900=CARTESIAN_POINT('',(0.,-1.55,-2.13));
#6901=CARTESIAN_POINT('',(-2.46585583768694,-1.55,-1.32648218523477));
#6902=CARTESIAN_POINT('Origin',(0.,-1.55,0.));
#6903=CARTESIAN_POINT('',(-1.68,-1.55,-0.84));
#6904=CARTESIAN_POINT('Origin',(-3.78,0.,-2.14));
#6905=CARTESIAN_POINT('',(-3.76384615384615,0.,-2.13));
#6906=CARTESIAN_POINT('',(-2.46585583768694,0.,-1.32648218523477));
#6907=CARTESIAN_POINT('Origin',(0.,-1.55,-1.49));
#6908=CARTESIAN_POINT('',(3.76384615384615,-1.55,-2.13));
#6909=CARTESIAN_POINT('',(1.81744325908679,-1.55,-2.13));
#6910=CARTESIAN_POINT('',(0.,-1.55,-2.13));
#6911=CARTESIAN_POINT('',(2.46585583768694,-1.55,-1.32648218523477));
#6912=CARTESIAN_POINT('',(3.78,-1.55,-2.14));
#6913=CARTESIAN_POINT('Origin',(0.,-1.55,0.));
#6914=CARTESIAN_POINT('Origin',(1.68,0.,-0.84));
#6915=CARTESIAN_POINT('',(3.76384615384615,0.,-2.13));
#6916=CARTESIAN_POINT('',(2.46585583768694,0.,-1.32648218523477));
#6917=CARTESIAN_POINT('Origin',(0.,0.,-2.13));
#6918=CARTESIAN_POINT('',(-6.35,1.9,-2.13));
#6919=CARTESIAN_POINT('',(-6.35,-1.9,-2.13));
#6920=CARTESIAN_POINT('',(-6.35,1.9,-2.13));
#6921=CARTESIAN_POINT('',(6.35,-1.9,-2.13));
#6922=CARTESIAN_POINT('',(-6.35,-1.9,-2.13));
#6923=CARTESIAN_POINT('',(6.35,1.9,-2.13));
#6924=CARTESIAN_POINT('',(6.35,-1.9,-2.13));
#6925=CARTESIAN_POINT('',(6.35,1.9,-2.13));
#6926=CARTESIAN_POINT('',(4.1,7.9602041944578E-17,-2.13));
#6927=CARTESIAN_POINT('Origin',(4.75,0.,-2.13));
#6928=CARTESIAN_POINT('',(-5.4,7.9602041944578E-17,-2.13));
#6929=CARTESIAN_POINT('Origin',(-4.75,0.,-2.13));
#6930=CARTESIAN_POINT('',(1.81744325908679,-1.65,-2.13));
#6931=CARTESIAN_POINT('',(1.81744325908679,0.,-2.13));
#6932=CARTESIAN_POINT('',(-1.81744325908679,-1.65,-2.13));
#6933=CARTESIAN_POINT('',(0.,-1.65,-2.13));
#6934=CARTESIAN_POINT('',(-1.81744325908679,0.,-2.13));
#6935=CARTESIAN_POINT('',(-1.81744325908679,1.65,-2.13));
#6936=CARTESIAN_POINT('',(-1.81744325908679,0.,-2.13));
#6937=CARTESIAN_POINT('',(1.81744325908679,1.65,-2.13));
#6938=CARTESIAN_POINT('',(0.,1.65,-2.13));
#6939=CARTESIAN_POINT('',(1.81744325908679,0.,-2.13));
#6940=CARTESIAN_POINT('Origin',(0.,0.,0.));
#6941=CARTESIAN_POINT('Origin',(0.,1.65,0.));
#6942=CARTESIAN_POINT('Origin',(0.,-1.65,0.));
#6943=CARTESIAN_POINT('Origin',(0.,-1.65,0.));
#6944=CARTESIAN_POINT('Origin',(0.,1.65,0.));
#6945=CARTESIAN_POINT('Origin',(3.35,1.4,-3.33));
#6946=CARTESIAN_POINT('',(3.35,1.4,-3.33));
#6947=CARTESIAN_POINT('',(-3.35,1.4,-3.33));
#6948=CARTESIAN_POINT('',(1.675,1.4,-3.33));
#6949=CARTESIAN_POINT('',(3.35,1.4,-2.83));
#6950=CARTESIAN_POINT('',(3.35,1.4,-3.33));
#6951=CARTESIAN_POINT('',(-3.35,1.4,-2.83));
#6952=CARTESIAN_POINT('',(3.35,1.4,-2.83));
#6953=CARTESIAN_POINT('',(-3.35,1.4,-3.33));
#6954=CARTESIAN_POINT('Origin',(3.35,-1.4,-3.33));
#6955=CARTESIAN_POINT('',(3.35,-1.4,-3.33));
#6956=CARTESIAN_POINT('',(3.35,-0.7,-3.33));
#6957=CARTESIAN_POINT('',(3.35,-1.4,-2.83));
#6958=CARTESIAN_POINT('',(3.35,-1.4,-3.33));
#6959=CARTESIAN_POINT('',(3.35,-1.4,-2.83));
#6960=CARTESIAN_POINT('Origin',(-3.35,-1.4,-3.33));
#6961=CARTESIAN_POINT('',(-3.35,-1.4,-3.33));
#6962=CARTESIAN_POINT('',(-1.675,-1.4,-3.33));
#6963=CARTESIAN_POINT('',(-3.35,-1.4,-2.83));
#6964=CARTESIAN_POINT('',(-3.35,-1.4,-3.33));
#6965=CARTESIAN_POINT('',(-3.35,-1.4,-2.83));
#6966=CARTESIAN_POINT('Origin',(-3.35,1.4,-3.33));
#6967=CARTESIAN_POINT('',(-3.35,0.7,-3.33));
#6968=CARTESIAN_POINT('',(-3.35,1.4,-2.83));
#6969=CARTESIAN_POINT('Origin',(0.,0.,-2.83));
#6970=CARTESIAN_POINT('Origin',(-4.75,0.,-3.33));
#6971=CARTESIAN_POINT('',(-5.4,-7.9602041944578E-17,-3.33));
#6972=CARTESIAN_POINT('Origin',(-4.75,0.,-3.33));
#6973=CARTESIAN_POINT('',(-5.4,-7.9602041944578E-17,-3.33));
#6974=CARTESIAN_POINT('Origin',(4.75,0.,-3.33));
#6975=CARTESIAN_POINT('',(4.1,-7.9602041944578E-17,-3.33));
#6976=CARTESIAN_POINT('Origin',(4.75,0.,-3.33));
#6977=CARTESIAN_POINT('',(4.1,-7.9602041944578E-17,-3.33));
#6978=CARTESIAN_POINT('Origin',(6.35,1.9,-3.33));
#6979=CARTESIAN_POINT('',(6.35,1.9,-3.33));
#6980=CARTESIAN_POINT('',(-6.35,1.9,-3.33));
#6981=CARTESIAN_POINT('',(6.35,1.9,-3.33));
#6982=CARTESIAN_POINT('',(-6.35,1.9,-3.33));
#6983=CARTESIAN_POINT('',(6.35,1.9,-3.33));
#6984=CARTESIAN_POINT('Origin',(6.35,-1.9,-3.33));
#6985=CARTESIAN_POINT('',(6.35,-1.9,-3.33));
#6986=CARTESIAN_POINT('',(6.35,-1.9,-3.33));
#6987=CARTESIAN_POINT('',(6.35,-1.9,-3.33));
#6988=CARTESIAN_POINT('Origin',(-6.35,-1.9,-3.33));
#6989=CARTESIAN_POINT('',(-6.35,-1.9,-3.33));
#6990=CARTESIAN_POINT('',(-6.35,-1.9,-3.33));
#6991=CARTESIAN_POINT('',(-6.35,-1.9,-3.33));
#6992=CARTESIAN_POINT('Origin',(-6.35,1.9,-3.33));
#6993=CARTESIAN_POINT('',(-6.35,1.9,-3.33));
#6994=CARTESIAN_POINT('Origin',(0.,0.,-3.33));
#8330=UNCERTAINTY_MEASURE_WITH_UNIT(LENGTH_MEASURE(0.001),#8378,
'DISTANCE_ACCURACY_VALUE',
'Maximum model space distance between geometric entities at asserted c
onnectivities');
#8345=UNCERTAINTY_MEASURE_WITH_UNIT(LENGTH_MEASURE(0.001),#8378,
'DISTANCE_ACCURACY_VALUE',
'Maximum model space distance between geometric entities at asserted c
onnectivities');
#8362=(
GEOMETRIC_REPRESENTATION_CONTEXT(3)
GLOBAL_UNCERTAINTY_ASSIGNED_CONTEXT((#8330))
GLOBAL_UNIT_ASSIGNED_CONTEXT((#8378,#8380,#8381))
REPRESENTATION_CONTEXT('','3D')
);
#8377=(
GEOMETRIC_REPRESENTATION_CONTEXT(3)
GLOBAL_UNCERTAINTY_ASSIGNED_CONTEXT((#8345))
GLOBAL_UNIT_ASSIGNED_CONTEXT((#8378,#8380,#8381))
REPRESENTATION_CONTEXT('','3D')
);
#8378=(
LENGTH_UNIT()
NAMED_UNIT(*)
SI_UNIT(.CENTI.,.METRE.)
);
#8380=(
NAMED_UNIT(*)
PLANE_ANGLE_UNIT()
SI_UNIT($,.RADIAN.)
);
#8381=(
NAMED_UNIT(*)
SI_UNIT($,.STERADIAN.)
SOLID_ANGLE_UNIT()
);
#8398=SHAPE_DEFINITION_REPRESENTATION(#8429,#8513);
#8429=PRODUCT_DEFINITION_SHAPE('',$,#8545);
#8513=SHAPE_REPRESENTATION('',(#4826),#8362);
#8528=PRODUCT_DEFINITION_CONTEXT('part definition',#8623,'design');
#8545=PRODUCT_DEFINITION('Housing','Housing',#8576,#8528);
#8576=PRODUCT_DEFINITION_FORMATION('',$,#8641);
#8623=APPLICATION_CONTEXT(
'Core Data for Automotive Mechanical Design Process');
#8624=PRODUCT_CONTEXT('part definition',#8623,'mechanical');
#8641=PRODUCT('Housing','Housing','Housing',(#8624));
#8691=COLOUR_RGB('Dark Blue',0.08,0.2,0.34);
#8692=FILL_AREA_STYLE_COLOUR('',#8691);
#8693=FILL_AREA_STYLE('',(#8692));
#8694=SURFACE_STYLE_FILL_AREA(#8693);
#8695=SURFACE_SIDE_STYLE('',(#8694));
#8696=SURFACE_STYLE_USAGE(.BOTH.,#8695);
#8697=PRESENTATION_STYLE_ASSIGNMENT((#8696));
ENDSEC;
END-ISO-10303-21;
